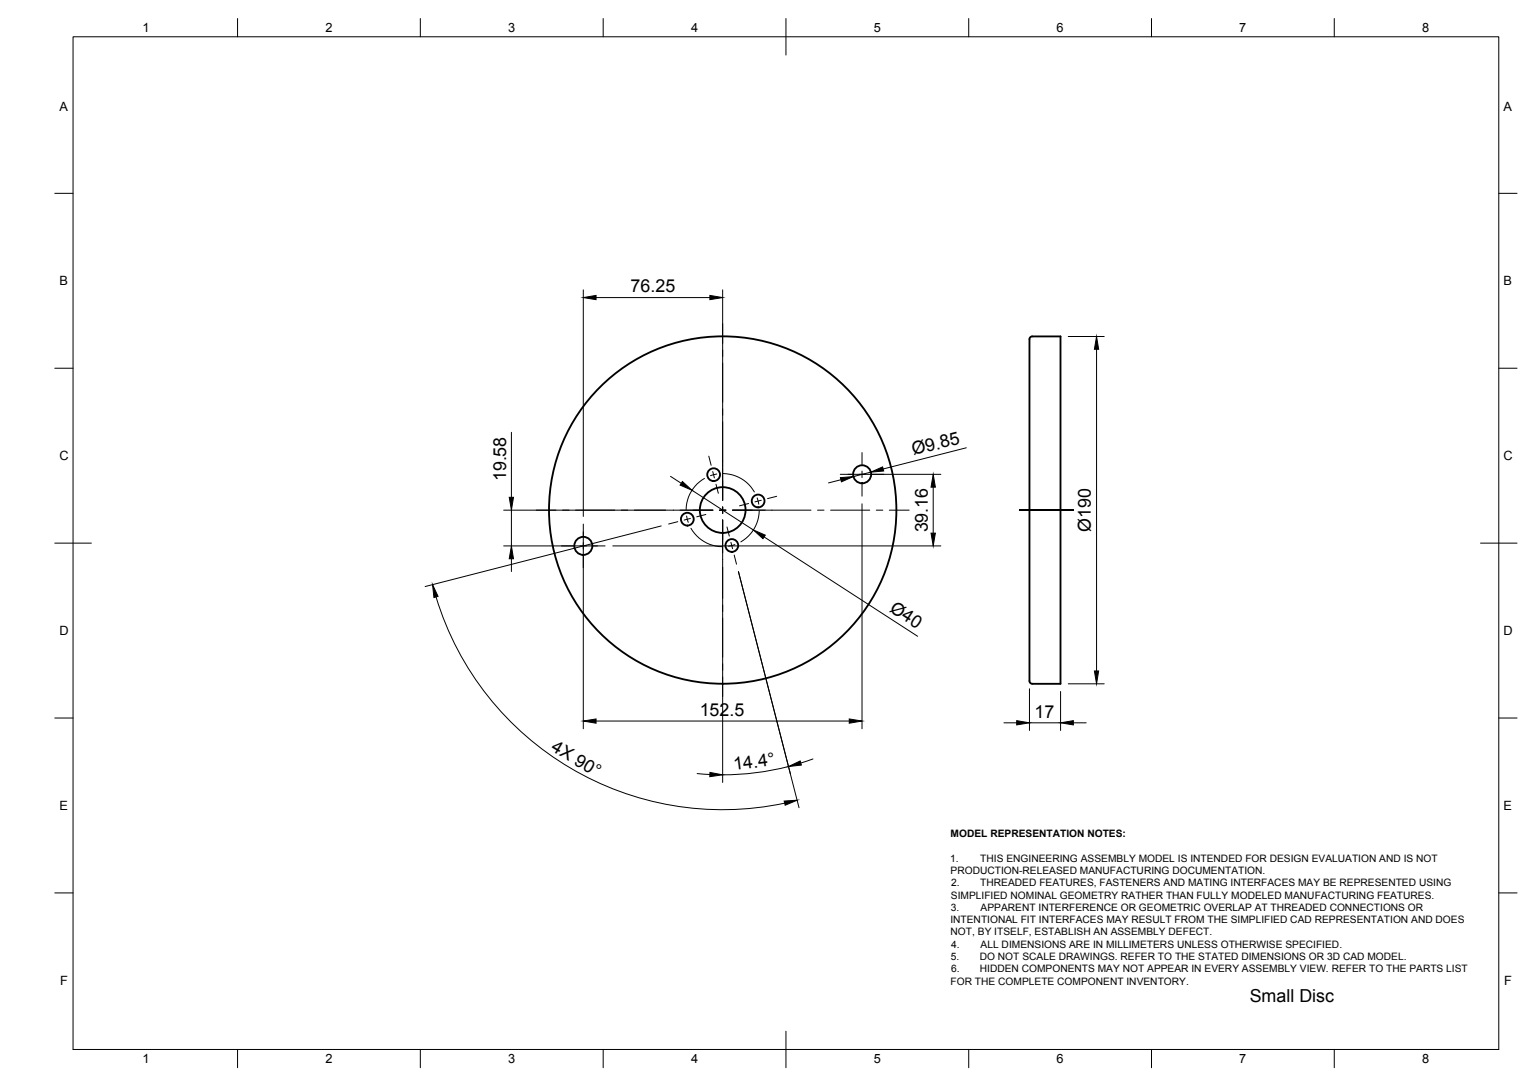
ISO-10303-21;
HEADER;
/* Generated by software containing ST-Developer
 * from STEP Tools, Inc. (www.steptools.com) 
 */

FILE_DESCRIPTION(
/* description */ ('STEP AP214'),
/* implementation_level */ '2;1');

FILE_NAME(
/* name */ 'SMALL DISC.step',
/* time_stamp */ '2026-10-06T11:20:11-07:00',
/* author */ (''),
/* organization */ (''),
/* preprocessor_version */ 'ST-DEVELOPER v20.2',
/* originating_system */ 'Autodesk Translation Framework v15.15.0.0',
/* authorisation */ '');

FILE_SCHEMA (('AUTOMOTIVE_DESIGN { 1 0 10303 214 3 1 1 }'));
ENDSEC;

DATA;
#10=MECHANICAL_DESIGN_GEOMETRIC_PRESENTATION_REPRESENTATION('',(#49),#2840);
#37=SHAPE_REPRESENTATION_RELATIONSHIP('SRR','None',#2868,#43);
#43=ADVANCED_BREP_SHAPE_REPRESENTATION('',(#55),#2836);
#49=STYLED_ITEM('',(#2905),#55);
#55=MANIFOLD_SOLID_BREP('Body1',#1549);
#68=TOROIDAL_SURFACE('',#1728,13.,0.5);
#69=TOROIDAL_SURFACE('',#1734,93.5,1.5);
#81=FACE_BOUND('',#275,.T.);
#82=FACE_BOUND('',#276,.T.);
#83=FACE_BOUND('',#277,.T.);
#84=FACE_BOUND('',#278,.T.);
#85=FACE_BOUND('',#279,.T.);
#86=FACE_BOUND('',#280,.T.);
#87=FACE_BOUND('',#281,.T.);
#88=FACE_BOUND('',#283,.T.);
#89=FACE_BOUND('',#284,.T.);
#90=FACE_BOUND('',#285,.T.);
#91=FACE_BOUND('',#286,.T.);
#92=FACE_BOUND('',#287,.T.);
#93=FACE_BOUND('',#288,.T.);
#94=FACE_BOUND('',#289,.T.);
#107=PLANE('',#1741);
#108=PLANE('',#1742);
#163=FACE_OUTER_BOUND('',#264,.T.);
#164=FACE_OUTER_BOUND('',#265,.T.);
#165=FACE_OUTER_BOUND('',#266,.T.);
#166=FACE_OUTER_BOUND('',#267,.T.);
#167=FACE_OUTER_BOUND('',#268,.T.);
#168=FACE_OUTER_BOUND('',#269,.T.);
#169=FACE_OUTER_BOUND('',#270,.T.);
#170=FACE_OUTER_BOUND('',#271,.T.);
#171=FACE_OUTER_BOUND('',#272,.T.);
#172=FACE_OUTER_BOUND('',#273,.T.);
#173=FACE_OUTER_BOUND('',#274,.T.);
#174=FACE_OUTER_BOUND('',#282,.T.);
#264=EDGE_LOOP('',(#1144,#1145,#1146,#1147));
#265=EDGE_LOOP('',(#1148,#1149,#1150,#1151));
#266=EDGE_LOOP('',(#1152,#1153,#1154,#1155));
#267=EDGE_LOOP('',(#1156,#1157,#1158,#1159));
#268=EDGE_LOOP('',(#1160,#1161,#1162,#1163));
#269=EDGE_LOOP('',(#1164,#1165,#1166,#1167));
#270=EDGE_LOOP('',(#1168,#1169,#1170,#1171));
#271=EDGE_LOOP('',(#1172,#1173,#1174,#1175));
#272=EDGE_LOOP('',(#1176,#1177,#1178,#1179,#1180));
#273=EDGE_LOOP('',(#1181,#1182,#1183,#1184,#1185));
#274=EDGE_LOOP('',(#1186));
#275=EDGE_LOOP('',(#1187));
#276=EDGE_LOOP('',(#1188));
#277=EDGE_LOOP('',(#1189));
#278=EDGE_LOOP('',(#1190));
#279=EDGE_LOOP('',(#1191));
#280=EDGE_LOOP('',(#1192));
#281=EDGE_LOOP('',(#1193));
#282=EDGE_LOOP('',(#1194));
#283=EDGE_LOOP('',(#1195));
#284=EDGE_LOOP('',(#1196));
#285=EDGE_LOOP('',(#1197));
#286=EDGE_LOOP('',(#1198));
#287=EDGE_LOOP('',(#1199));
#288=EDGE_LOOP('',(#1200));
#289=EDGE_LOOP('',(#1201));
#365=LINE('',#2549,#458);
#366=LINE('',#2555,#459);
#367=LINE('',#2561,#460);
#368=LINE('',#2567,#461);
#369=LINE('',#2573,#462);
#370=LINE('',#2579,#463);
#371=LINE('',#2590,#464);
#372=LINE('',#2602,#465);
#458=VECTOR('',#2056,4.92500000000001);
#459=VECTOR('',#2063,4.92500000000001);
#460=VECTOR('',#2070,3.5);
#461=VECTOR('',#2077,3.5);
#462=VECTOR('',#2084,3.5);
#463=VECTOR('',#2091,3.5);
#464=VECTOR('',#2106,12.5);
#465=VECTOR('',#2121,95.0000000000003);
#569=CIRCLE('',#1711,4.92500000000001);
#570=CIRCLE('',#1712,4.92500000000001);
#571=CIRCLE('',#1714,4.92500000000001);
#572=CIRCLE('',#1715,4.92500000000001);
#573=CIRCLE('',#1717,3.5);
#574=CIRCLE('',#1718,3.5);
#575=CIRCLE('',#1720,3.5);
#576=CIRCLE('',#1721,3.5);
#577=CIRCLE('',#1723,3.5);
#578=CIRCLE('',#1724,3.5);
#579=CIRCLE('',#1726,3.5);
#580=CIRCLE('',#1727,3.5);
#581=CIRCLE('',#1729,12.5000000000001);
#582=CIRCLE('',#1730,0.5);
#583=CIRCLE('',#1731,13.0000000000001);
#584=CIRCLE('',#1733,12.5000000000001);
#585=CIRCLE('',#1735,93.5000000000003);
#586=CIRCLE('',#1736,1.5);
#587=CIRCLE('',#1737,95.0000000000003);
#588=CIRCLE('',#1738,95.0000000000003);
#589=CIRCLE('',#1740,95.0000000000003);
#686=VERTEX_POINT('',#2546);
#687=VERTEX_POINT('',#2548);
#688=VERTEX_POINT('',#2552);
#689=VERTEX_POINT('',#2554);
#690=VERTEX_POINT('',#2558);
#691=VERTEX_POINT('',#2560);
#692=VERTEX_POINT('',#2564);
#693=VERTEX_POINT('',#2566);
#694=VERTEX_POINT('',#2570);
#695=VERTEX_POINT('',#2572);
#696=VERTEX_POINT('',#2576);
#697=VERTEX_POINT('',#2578);
#698=VERTEX_POINT('',#2582);
#699=VERTEX_POINT('',#2584);
#700=VERTEX_POINT('',#2588);
#701=VERTEX_POINT('',#2592);
#702=VERTEX_POINT('',#2594);
#703=VERTEX_POINT('',#2596);
#704=VERTEX_POINT('',#2600);
#853=EDGE_CURVE('',#686,#686,#569,.T.);
#854=EDGE_CURVE('',#686,#687,#365,.T.);
#855=EDGE_CURVE('',#687,#687,#570,.T.);
#856=EDGE_CURVE('',#688,#688,#571,.T.);
#857=EDGE_CURVE('',#688,#689,#366,.T.);
#858=EDGE_CURVE('',#689,#689,#572,.T.);
#859=EDGE_CURVE('',#690,#690,#573,.T.);
#860=EDGE_CURVE('',#690,#691,#367,.T.);
#861=EDGE_CURVE('',#691,#691,#574,.T.);
#862=EDGE_CURVE('',#692,#692,#575,.T.);
#863=EDGE_CURVE('',#692,#693,#368,.T.);
#864=EDGE_CURVE('',#693,#693,#576,.T.);
#865=EDGE_CURVE('',#694,#694,#577,.T.);
#866=EDGE_CURVE('',#694,#695,#369,.T.);
#867=EDGE_CURVE('',#695,#695,#578,.T.);
#868=EDGE_CURVE('',#696,#696,#579,.T.);
#869=EDGE_CURVE('',#696,#697,#370,.T.);
#870=EDGE_CURVE('',#697,#697,#580,.T.);
#871=EDGE_CURVE('',#698,#698,#581,.T.);
#872=EDGE_CURVE('',#698,#699,#582,.T.);
#873=EDGE_CURVE('',#699,#699,#583,.T.);
#874=EDGE_CURVE('',#700,#700,#584,.T.);
#875=EDGE_CURVE('',#700,#698,#371,.T.);
#876=EDGE_CURVE('',#701,#701,#585,.T.);
#877=EDGE_CURVE('',#701,#702,#586,.T.);
#878=EDGE_CURVE('',#703,#702,#587,.T.);
#879=EDGE_CURVE('',#702,#703,#588,.T.);
#880=EDGE_CURVE('',#704,#704,#589,.T.);
#881=EDGE_CURVE('',#704,#703,#372,.T.);
#1144=ORIENTED_EDGE('',*,*,#853,.F.);
#1145=ORIENTED_EDGE('',*,*,#854,.T.);
#1146=ORIENTED_EDGE('',*,*,#855,.T.);
#1147=ORIENTED_EDGE('',*,*,#854,.F.);
#1148=ORIENTED_EDGE('',*,*,#856,.F.);
#1149=ORIENTED_EDGE('',*,*,#857,.T.);
#1150=ORIENTED_EDGE('',*,*,#858,.T.);
#1151=ORIENTED_EDGE('',*,*,#857,.F.);
#1152=ORIENTED_EDGE('',*,*,#859,.F.);
#1153=ORIENTED_EDGE('',*,*,#860,.T.);
#1154=ORIENTED_EDGE('',*,*,#861,.T.);
#1155=ORIENTED_EDGE('',*,*,#860,.F.);
#1156=ORIENTED_EDGE('',*,*,#862,.F.);
#1157=ORIENTED_EDGE('',*,*,#863,.T.);
#1158=ORIENTED_EDGE('',*,*,#864,.T.);
#1159=ORIENTED_EDGE('',*,*,#863,.F.);
#1160=ORIENTED_EDGE('',*,*,#865,.F.);
#1161=ORIENTED_EDGE('',*,*,#866,.T.);
#1162=ORIENTED_EDGE('',*,*,#867,.T.);
#1163=ORIENTED_EDGE('',*,*,#866,.F.);
#1164=ORIENTED_EDGE('',*,*,#868,.F.);
#1165=ORIENTED_EDGE('',*,*,#869,.T.);
#1166=ORIENTED_EDGE('',*,*,#870,.T.);
#1167=ORIENTED_EDGE('',*,*,#869,.F.);
#1168=ORIENTED_EDGE('',*,*,#871,.F.);
#1169=ORIENTED_EDGE('',*,*,#872,.T.);
#1170=ORIENTED_EDGE('',*,*,#873,.F.);
#1171=ORIENTED_EDGE('',*,*,#872,.F.);
#1172=ORIENTED_EDGE('',*,*,#874,.F.);
#1173=ORIENTED_EDGE('',*,*,#875,.T.);
#1174=ORIENTED_EDGE('',*,*,#871,.T.);
#1175=ORIENTED_EDGE('',*,*,#875,.F.);
#1176=ORIENTED_EDGE('',*,*,#876,.F.);
#1177=ORIENTED_EDGE('',*,*,#877,.T.);
#1178=ORIENTED_EDGE('',*,*,#878,.F.);
#1179=ORIENTED_EDGE('',*,*,#879,.F.);
#1180=ORIENTED_EDGE('',*,*,#877,.F.);
#1181=ORIENTED_EDGE('',*,*,#880,.T.);
#1182=ORIENTED_EDGE('',*,*,#881,.T.);
#1183=ORIENTED_EDGE('',*,*,#878,.T.);
#1184=ORIENTED_EDGE('',*,*,#879,.T.);
#1185=ORIENTED_EDGE('',*,*,#881,.F.);
#1186=ORIENTED_EDGE('',*,*,#876,.T.);
#1187=ORIENTED_EDGE('',*,*,#855,.F.);
#1188=ORIENTED_EDGE('',*,*,#858,.F.);
#1189=ORIENTED_EDGE('',*,*,#861,.F.);
#1190=ORIENTED_EDGE('',*,*,#864,.F.);
#1191=ORIENTED_EDGE('',*,*,#867,.F.);
#1192=ORIENTED_EDGE('',*,*,#870,.F.);
#1193=ORIENTED_EDGE('',*,*,#873,.T.);
#1194=ORIENTED_EDGE('',*,*,#880,.F.);
#1195=ORIENTED_EDGE('',*,*,#853,.T.);
#1196=ORIENTED_EDGE('',*,*,#856,.T.);
#1197=ORIENTED_EDGE('',*,*,#859,.T.);
#1198=ORIENTED_EDGE('',*,*,#862,.T.);
#1199=ORIENTED_EDGE('',*,*,#865,.T.);
#1200=ORIENTED_EDGE('',*,*,#868,.T.);
#1201=ORIENTED_EDGE('',*,*,#874,.T.);
#1425=CYLINDRICAL_SURFACE('',#1710,4.92500000000001);
#1426=CYLINDRICAL_SURFACE('',#1713,4.92500000000001);
#1427=CYLINDRICAL_SURFACE('',#1716,3.5);
#1428=CYLINDRICAL_SURFACE('',#1719,3.5);
#1429=CYLINDRICAL_SURFACE('',#1722,3.5);
#1430=CYLINDRICAL_SURFACE('',#1725,3.5);
#1431=CYLINDRICAL_SURFACE('',#1732,12.5);
#1432=CYLINDRICAL_SURFACE('',#1739,95.0000000000003);
#1494=ADVANCED_FACE('',(#163),#1425,.F.);
#1495=ADVANCED_FACE('',(#164),#1426,.F.);
#1496=ADVANCED_FACE('',(#165),#1427,.F.);
#1497=ADVANCED_FACE('',(#166),#1428,.F.);
#1498=ADVANCED_FACE('',(#167),#1429,.F.);
#1499=ADVANCED_FACE('',(#168),#1430,.F.);
#1500=ADVANCED_FACE('',(#169),#68,.T.);
#1501=ADVANCED_FACE('',(#170),#1431,.F.);
#1502=ADVANCED_FACE('',(#171),#69,.T.);
#1503=ADVANCED_FACE('',(#172),#1432,.T.);
#1504=ADVANCED_FACE('',(#173,#81,#82,#83,#84,#85,#86,#87),#107,.T.);
#1505=ADVANCED_FACE('',(#174,#88,#89,#90,#91,#92,#93,#94),#108,.F.);
#1549=CLOSED_SHELL('',(#1494,#1495,#1496,#1497,#1498,#1499,#1500,#1501,
#1502,#1503,#1504,#1505));
#1709=AXIS2_PLACEMENT_3D('',#2544,#2050,#2051);
#1710=AXIS2_PLACEMENT_3D('',#2545,#2052,#2053);
#1711=AXIS2_PLACEMENT_3D('',#2547,#2054,#2055);
#1712=AXIS2_PLACEMENT_3D('',#2550,#2057,#2058);
#1713=AXIS2_PLACEMENT_3D('',#2551,#2059,#2060);
#1714=AXIS2_PLACEMENT_3D('',#2553,#2061,#2062);
#1715=AXIS2_PLACEMENT_3D('',#2556,#2064,#2065);
#1716=AXIS2_PLACEMENT_3D('',#2557,#2066,#2067);
#1717=AXIS2_PLACEMENT_3D('',#2559,#2068,#2069);
#1718=AXIS2_PLACEMENT_3D('',#2562,#2071,#2072);
#1719=AXIS2_PLACEMENT_3D('',#2563,#2073,#2074);
#1720=AXIS2_PLACEMENT_3D('',#2565,#2075,#2076);
#1721=AXIS2_PLACEMENT_3D('',#2568,#2078,#2079);
#1722=AXIS2_PLACEMENT_3D('',#2569,#2080,#2081);
#1723=AXIS2_PLACEMENT_3D('',#2571,#2082,#2083);
#1724=AXIS2_PLACEMENT_3D('',#2574,#2085,#2086);
#1725=AXIS2_PLACEMENT_3D('',#2575,#2087,#2088);
#1726=AXIS2_PLACEMENT_3D('',#2577,#2089,#2090);
#1727=AXIS2_PLACEMENT_3D('',#2580,#2092,#2093);
#1728=AXIS2_PLACEMENT_3D('',#2581,#2094,#2095);
#1729=AXIS2_PLACEMENT_3D('',#2583,#2096,#2097);
#1730=AXIS2_PLACEMENT_3D('',#2585,#2098,#2099);
#1731=AXIS2_PLACEMENT_3D('',#2586,#2100,#2101);
#1732=AXIS2_PLACEMENT_3D('',#2587,#2102,#2103);
#1733=AXIS2_PLACEMENT_3D('',#2589,#2104,#2105);
#1734=AXIS2_PLACEMENT_3D('',#2591,#2107,#2108);
#1735=AXIS2_PLACEMENT_3D('',#2593,#2109,#2110);
#1736=AXIS2_PLACEMENT_3D('',#2595,#2111,#2112);
#1737=AXIS2_PLACEMENT_3D('',#2597,#2113,#2114);
#1738=AXIS2_PLACEMENT_3D('',#2598,#2115,#2116);
#1739=AXIS2_PLACEMENT_3D('',#2599,#2117,#2118);
#1740=AXIS2_PLACEMENT_3D('',#2601,#2119,#2120);
#1741=AXIS2_PLACEMENT_3D('',#2603,#2122,#2123);
#1742=AXIS2_PLACEMENT_3D('',#2604,#2124,#2125);
#2050=DIRECTION('axis',(0.,0.,1.));
#2051=DIRECTION('refdir',(1.,0.,0.));
#2052=DIRECTION('center_axis',(-5.42341872339446E-30,1.,2.7856650715617E-30));
#2053=DIRECTION('ref_axis',(1.51078281062137E-59,-2.7856650715617E-30,1.));
#2054=DIRECTION('center_axis',(-5.42341872339446E-30,1.,2.7856650715617E-30));
#2055=DIRECTION('ref_axis',(2.8681187888985E-59,-2.7856650715617E-30,1.));
#2056=DIRECTION('',(-5.42341872339446E-30,1.,2.7856650715617E-30));
#2057=DIRECTION('center_axis',(-5.42341872339446E-30,1.,2.7856650715617E-30));
#2058=DIRECTION('ref_axis',(1.51078281062137E-59,-2.7856650715617E-30,1.));
#2059=DIRECTION('center_axis',(-5.42341872339446E-30,1.,2.7856650715617E-30));
#2060=DIRECTION('ref_axis',(1.51078281062137E-59,-2.7856650715617E-30,1.));
#2061=DIRECTION('center_axis',(-5.42341872339446E-30,1.,2.7856650715617E-30));
#2062=DIRECTION('ref_axis',(3.02156562124273E-59,-2.7856650715617E-30,1.));
#2063=DIRECTION('',(-5.42341872339446E-30,1.,2.7856650715617E-30));
#2064=DIRECTION('center_axis',(-5.42341872339446E-30,1.,2.7856650715617E-30));
#2065=DIRECTION('ref_axis',(1.51078281062137E-59,-2.7856650715617E-30,1.));
#2066=DIRECTION('center_axis',(-5.42341872339446E-30,1.,2.7856650715617E-30));
#2067=DIRECTION('ref_axis',(1.51078281062137E-59,-2.7856650715617E-30,1.));
#2068=DIRECTION('center_axis',(-5.42341872339446E-30,1.,2.7856650715617E-30));
#2069=DIRECTION('ref_axis',(3.02156562124273E-59,-2.7856650715617E-30,1.));
#2070=DIRECTION('',(-5.42341872339446E-30,1.,2.7856650715617E-30));
#2071=DIRECTION('center_axis',(-5.42341872339446E-30,1.,2.7856650715617E-30));
#2072=DIRECTION('ref_axis',(1.51078281062137E-59,-2.7856650715617E-30,1.));
#2073=DIRECTION('center_axis',(-5.42341872339446E-30,1.,2.7856650715617E-30));
#2074=DIRECTION('ref_axis',(1.51078281062137E-59,-2.7856650715617E-30,1.));
#2075=DIRECTION('center_axis',(-5.42341872339446E-30,1.,2.7856650715617E-30));
#2076=DIRECTION('ref_axis',(3.02156562124273E-59,-2.7856650715617E-30,1.));
#2077=DIRECTION('',(-5.42341872339446E-30,1.,2.7856650715617E-30));
#2078=DIRECTION('center_axis',(-5.42341872339446E-30,1.,2.7856650715617E-30));
#2079=DIRECTION('ref_axis',(1.51078281062137E-59,-2.7856650715617E-30,1.));
#2080=DIRECTION('center_axis',(-5.42341872339446E-30,1.,2.7856650715617E-30));
#2081=DIRECTION('ref_axis',(1.51078281062137E-59,-2.7856650715617E-30,1.));
#2082=DIRECTION('center_axis',(-5.42341872339446E-30,1.,2.7856650715617E-30));
#2083=DIRECTION('ref_axis',(3.02156562124273E-59,-2.7856650715617E-30,1.));
#2084=DIRECTION('',(-5.42341872339446E-30,1.,2.7856650715617E-30));
#2085=DIRECTION('center_axis',(-5.42341872339446E-30,1.,2.7856650715617E-30));
#2086=DIRECTION('ref_axis',(1.51078281062137E-59,-2.7856650715617E-30,1.));
#2087=DIRECTION('center_axis',(-5.42341872339446E-30,1.,2.7856650715617E-30));
#2088=DIRECTION('ref_axis',(1.51078281062137E-59,-2.7856650715617E-30,1.));
#2089=DIRECTION('center_axis',(-5.42341872339446E-30,1.,2.7856650715617E-30));
#2090=DIRECTION('ref_axis',(3.02156562124273E-59,-2.7856650715617E-30,1.));
#2091=DIRECTION('',(-5.42341872339446E-30,1.,2.7856650715617E-30));
#2092=DIRECTION('center_axis',(-5.42341872339446E-30,1.,2.7856650715617E-30));
#2093=DIRECTION('ref_axis',(1.51078281062137E-59,-2.7856650715617E-30,1.));
#2094=DIRECTION('center_axis',(-5.42341872339446E-30,1.,2.7856650715617E-30));
#2095=DIRECTION('ref_axis',(0.,0.,1.));
#2096=DIRECTION('center_axis',(-5.42341872339446E-30,1.,2.7856650715617E-30));
#2097=DIRECTION('ref_axis',(1.51078281062137E-59,-2.7856650715617E-30,1.));
#2098=DIRECTION('center_axis',(-1.,-5.42341872339446E-30,1.64477485129653E-16));
#2099=DIRECTION('ref_axis',(-1.64477485129653E-16,0.,-1.));
#2100=DIRECTION('center_axis',(5.42341872339446E-30,-1.,-2.7856650715617E-30));
#2101=DIRECTION('ref_axis',(1.51078281062137E-59,-2.7856650715617E-30,1.));
#2102=DIRECTION('center_axis',(-5.42341872339446E-30,1.,3.00753220115511E-30));
#2103=DIRECTION('ref_axis',(1.63111064509564E-59,-3.00753220115511E-30,
1.));
#2104=DIRECTION('center_axis',(-5.42341872339446E-30,1.,2.7856650715617E-30));
#2105=DIRECTION('ref_axis',(3.02156562124273E-59,-2.7856650715617E-30,1.));
#2106=DIRECTION('',(-5.42341872339446E-30,1.,3.00753220115511E-30));
#2107=DIRECTION('center_axis',(-5.42341872339446E-30,1.,2.7856650715617E-30));
#2108=DIRECTION('ref_axis',(3.73969860926369E-17,0.,1.));
#2109=DIRECTION('center_axis',(-5.42341872339446E-30,1.,2.7856650715617E-30));
#2110=DIRECTION('ref_axis',(3.71063845128728E-17,-2.7856650715617E-30,1.));
#2111=DIRECTION('center_axis',(-1.,-5.42341872339446E-30,1.63611814155286E-16));
#2112=DIRECTION('ref_axis',(-1.63611814155286E-16,0.,-1.));
#2113=DIRECTION('center_axis',(5.42341872339446E-30,-1.,-2.7856650715617E-30));
#2114=DIRECTION('ref_axis',(3.65204942310906E-17,-2.7856650715617E-30,1.));
#2115=DIRECTION('center_axis',(5.42341872339446E-30,-1.,-2.7856650715617E-30));
#2116=DIRECTION('ref_axis',(3.65204942310906E-17,-2.7856650715617E-30,1.));
#2117=DIRECTION('center_axis',(5.42341872339446E-30,-1.,-2.7856650715617E-30));
#2118=DIRECTION('ref_axis',(-3.65204942310906E-17,2.7856650715617E-30,-1.));
#2119=DIRECTION('center_axis',(-5.42341872339446E-30,1.,2.7856650715617E-30));
#2120=DIRECTION('ref_axis',(3.65204942310906E-17,-2.7856650715617E-30,1.));
#2121=DIRECTION('',(-5.42341872339446E-30,1.,2.7856650715617E-30));
#2122=DIRECTION('center_axis',(-5.42341872339446E-30,1.,-2.78566507156169E-30));
#2123=DIRECTION('ref_axis',(2.77555756156288E-17,2.78566507156169E-30,1.));
#2124=DIRECTION('center_axis',(-5.42341872339446E-30,1.,-2.78566507156169E-30));
#2125=DIRECTION('ref_axis',(2.77555756156288E-17,2.78566507156169E-30,1.));
#2544=CARTESIAN_POINT('',(0.,0.,0.));
#2545=CARTESIAN_POINT('Origin',(97.46416980426,17.,303.733119632278));
#2546=CARTESIAN_POINT('',(97.46416980426,4.88498130835069E-14,298.808119632278));
#2547=CARTESIAN_POINT('Origin',(97.46416980426,4.85722573273506E-14,303.733119632278));
#2548=CARTESIAN_POINT('',(97.46416980426,17.,298.808119632278));
#2549=CARTESIAN_POINT('',(97.46416980426,17.,298.808119632278));
#2550=CARTESIAN_POINT('Origin',(97.46416980426,17.,303.733119632278));
#2551=CARTESIAN_POINT('Origin',(-59.9821245185343,17.,303.733119632278));
#2552=CARTESIAN_POINT('',(-59.9821245185343,0.,298.808119632278));
#2553=CARTESIAN_POINT('Origin',(-59.9821245185343,0.,303.733119632278));
#2554=CARTESIAN_POINT('',(-59.9821245185343,17.,298.808119632278));
#2555=CARTESIAN_POINT('',(-59.9821245185343,17.,298.808119632278));
#2556=CARTESIAN_POINT('Origin',(-59.9821245185343,17.,303.733119632278));
#2557=CARTESIAN_POINT('Origin',(18.741022642863,17.,283.733119632278));
#2558=CARTESIAN_POINT('',(18.741022642863,0.,280.233119632278));
#2559=CARTESIAN_POINT('Origin',(18.7410226428626,0.,283.733119632278));
#2560=CARTESIAN_POINT('',(18.741022642863,17.,280.233119632278));
#2561=CARTESIAN_POINT('',(18.741022642863,17.,280.233119632278));
#2562=CARTESIAN_POINT('Origin',(18.741022642863,17.,283.733119632278));
#2563=CARTESIAN_POINT('Origin',(38.7410226428653,17.,303.733119632278));
#2564=CARTESIAN_POINT('',(38.7410226428653,0.,300.233119632278));
#2565=CARTESIAN_POINT('Origin',(38.7410226428657,0.,303.733119632278));
#2566=CARTESIAN_POINT('',(38.7410226428653,17.,300.233119632278));
#2567=CARTESIAN_POINT('',(38.7410226428653,17.,300.233119632278));
#2568=CARTESIAN_POINT('Origin',(38.7410226428653,17.,303.733119632278));
#2569=CARTESIAN_POINT('Origin',(18.7410226428626,17.,323.733119632279));
#2570=CARTESIAN_POINT('',(18.7410226428626,0.,320.233119632279));
#2571=CARTESIAN_POINT('Origin',(18.7410226428626,0.,323.733119632278));
#2572=CARTESIAN_POINT('',(18.7410226428626,17.,320.233119632279));
#2573=CARTESIAN_POINT('',(18.7410226428626,17.,320.233119632279));
#2574=CARTESIAN_POINT('Origin',(18.7410226428626,17.,323.733119632279));
#2575=CARTESIAN_POINT('Origin',(-1.25897735713698,17.,303.733119632279));
#2576=CARTESIAN_POINT('',(-1.25897735713698,0.,300.233119632279));
#2577=CARTESIAN_POINT('Origin',(-1.25897735713698,0.,303.733119632279));
#2578=CARTESIAN_POINT('',(-1.25897735713698,17.,300.233119632279));
#2579=CARTESIAN_POINT('',(-1.25897735713698,17.,300.233119632279));
#2580=CARTESIAN_POINT('Origin',(-1.25897735713698,17.,303.733119632279));
#2581=CARTESIAN_POINT('Origin',(18.7410226428648,16.5,303.733119632278));
#2582=CARTESIAN_POINT('',(18.7410226428648,16.5,291.233119632278));
#2583=CARTESIAN_POINT('Origin',(18.7410226428648,16.5,303.733119632278));
#2584=CARTESIAN_POINT('',(18.7410226428648,17.,290.733119632278));
#2585=CARTESIAN_POINT('Origin',(18.7410226428648,16.5,290.733119632278));
#2586=CARTESIAN_POINT('Origin',(18.7410226428648,17.,303.733119632278));
#2587=CARTESIAN_POINT('Origin',(18.7410226428644,-73.,303.733119632278));
#2588=CARTESIAN_POINT('',(18.7410226428644,0.,291.233119632278));
#2589=CARTESIAN_POINT('Origin',(18.7410226428644,0.,303.733119632278));
#2590=CARTESIAN_POINT('',(18.7410226428644,-73.,291.233119632278));
#2591=CARTESIAN_POINT('Origin',(18.7410226428648,15.5,303.733119632278));
#2592=CARTESIAN_POINT('',(18.7410226428648,17.,210.233119632278));
#2593=CARTESIAN_POINT('Origin',(18.7410226428648,17.,303.733119632278));
#2594=CARTESIAN_POINT('',(18.7410226428648,15.5,208.733119632278));
#2595=CARTESIAN_POINT('Origin',(18.7410226428648,15.5,210.233119632278));
#2596=CARTESIAN_POINT('',(18.7410226428648,15.5,398.733119632278));
#2597=CARTESIAN_POINT('Origin',(18.7410226428648,15.5,303.733119632278));
#2598=CARTESIAN_POINT('Origin',(18.7410226428648,15.5,303.733119632278));
#2599=CARTESIAN_POINT('Origin',(18.7410226428648,17.,303.733119632278));
#2600=CARTESIAN_POINT('',(18.7410226428648,-2.22044604925031E-15,398.733119632279));
#2601=CARTESIAN_POINT('Origin',(18.7410226428644,0.,303.733119632278));
#2602=CARTESIAN_POINT('',(18.7410226428648,17.,398.733119632279));
#2603=CARTESIAN_POINT('Origin',(18.7410226428648,17.,303.733119632278));
#2604=CARTESIAN_POINT('Origin',(18.7410226428644,0.,303.733119632278));
#2828=UNCERTAINTY_MEASURE_WITH_UNIT(LENGTH_MEASURE(0.01),#2841,
'DISTANCE_ACCURACY_VALUE',
'Maximum model space distance between geometric entities at asserted c
onnectivities');
#2832=UNCERTAINTY_MEASURE_WITH_UNIT(LENGTH_MEASURE(0.01),#2841,
'DISTANCE_ACCURACY_VALUE',
'Maximum model space distance between geometric entities at asserted c
onnectivities');
#2836=(
GEOMETRIC_REPRESENTATION_CONTEXT(3)
GLOBAL_UNCERTAINTY_ASSIGNED_CONTEXT((#2828))
GLOBAL_UNIT_ASSIGNED_CONTEXT((#2841,#2843,#2844))
REPRESENTATION_CONTEXT('','3D')
);
#2840=(
GEOMETRIC_REPRESENTATION_CONTEXT(3)
GLOBAL_UNCERTAINTY_ASSIGNED_CONTEXT((#2832))
GLOBAL_UNIT_ASSIGNED_CONTEXT((#2841,#2843,#2844))
REPRESENTATION_CONTEXT('','3D')
);
#2841=(
LENGTH_UNIT()
NAMED_UNIT(*)
SI_UNIT(.MILLI.,.METRE.)
);
#2843=(
NAMED_UNIT(*)
PLANE_ANGLE_UNIT()
SI_UNIT($,.RADIAN.)
);
#2844=(
NAMED_UNIT(*)
SI_UNIT($,.STERADIAN.)
SOLID_ANGLE_UNIT()
);
#2848=SHAPE_DEFINITION_REPRESENTATION(#2855,#2868);
#2855=PRODUCT_DEFINITION_SHAPE('',$,#2876);
#2868=SHAPE_REPRESENTATION('',(#1709),#2836);
#2872=PRODUCT_DEFINITION_CONTEXT('part definition',#2895,'design');
#2876=PRODUCT_DEFINITION('SMALL DISC','SMALL DISC',#2883,#2872);
#2883=PRODUCT_DEFINITION_FORMATION('',$,#2900);
#2895=APPLICATION_CONTEXT(
'Core Data for Automotive Mechanical Design Process');
#2896=PRODUCT_CONTEXT('part definition',#2895,'mechanical');
#2900=PRODUCT('SMALL DISC','SMALL DISC',$,(#2896));
#2905=PRESENTATION_STYLE_ASSIGNMENT((#2907));
#2907=SURFACE_STYLE_USAGE(.BOTH.,#2909);
#2909=SURFACE_SIDE_STYLE('',(#2911));
#2911=SURFACE_STYLE_FILL_AREA(#2913);
#2913=FILL_AREA_STYLE('Opaque(202,209,238)',(#2915));
#2915=FILL_AREA_STYLE_COLOUR('Opaque(202,209,238)',#2917);
#2917=COLOUR_RGB('Opaque(202,209,238)', 0.66274510, 0.83137255, 0.94901961);
ENDSEC;
END-ISO-10303-21;
